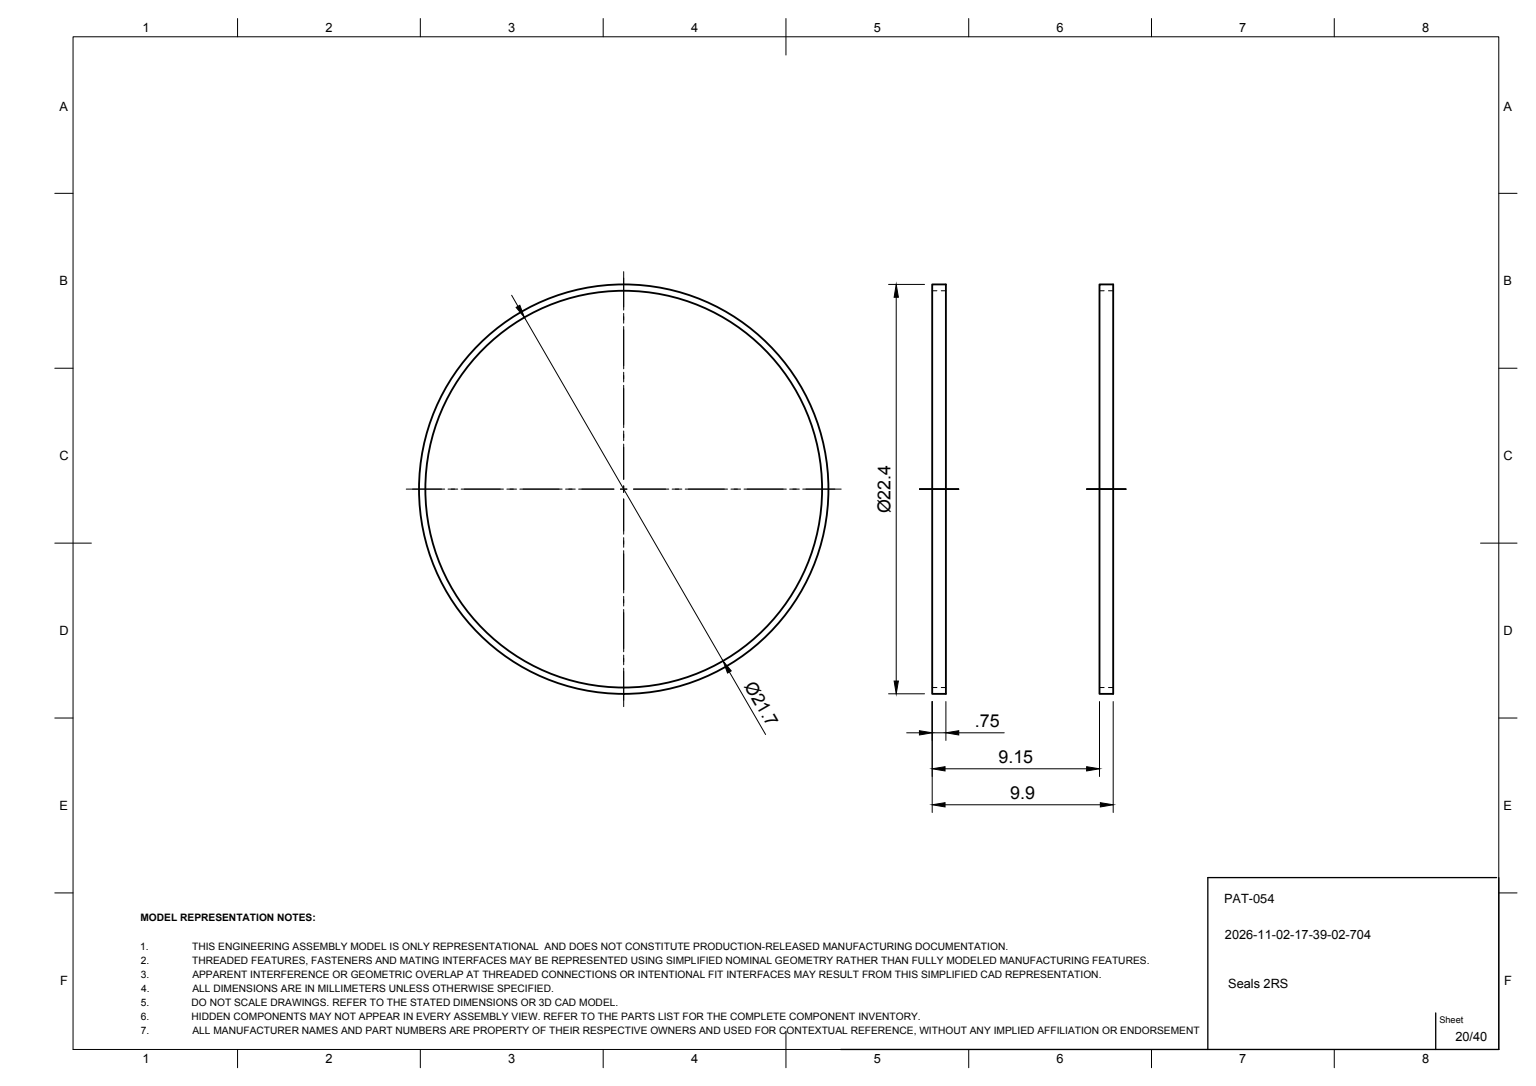
ISO-10303-21;
HEADER;
/* Generated by software containing ST-Developer
 * from STEP Tools, Inc. (www.steptools.com) 
 */

FILE_DESCRIPTION(
/* description */ ('PAT-054'),
/* implementation_level */ '2;1');

FILE_NAME(
/* name */ 'Seals 2RS.step',
/* time_stamp */ '2026-10-29T16:38:13-07:00',
/* author */ (''),
/* organization */ (''),
/* preprocessor_version */ 'ST-DEVELOPER v20.2',
/* originating_system */ 'Autodesk Translation Framework v15.17.0.0',
/* authorisation */ '');

FILE_SCHEMA (('AUTOMOTIVE_DESIGN { 1 0 10303 214 3 1 1 }'));
ENDSEC;

DATA;
#10=MECHANICAL_DESIGN_GEOMETRIC_PRESENTATION_REPRESENTATION('',(#918,#919),#33981);
#824=SHAPE_REPRESENTATION_RELATIONSHIP('SRR','None',#34198,#868);
#868=ADVANCED_BREP_SHAPE_REPRESENTATION('',(#977,#978),#33946);
#918=STYLED_ITEM('',(#34517),#977);
#919=STYLED_ITEM('',(#34517),#978);
#977=MANIFOLD_SOLID_BREP('Body1',#13029);
#978=MANIFOLD_SOLID_BREP('Body2',#13030);
#1133=FACE_BOUND('',#2613,.T.);
#1134=FACE_BOUND('',#2616,.T.);
#1135=FACE_BOUND('',#2619,.T.);
#1136=FACE_BOUND('',#2622,.T.);
#1323=PLANE('',#13978);
#1324=PLANE('',#13983);
#1325=PLANE('',#13986);
#1326=PLANE('',#13991);
#1768=FACE_OUTER_BOUND('',#2612,.T.);
#1769=FACE_OUTER_BOUND('',#2614,.T.);
#1770=FACE_OUTER_BOUND('',#2615,.T.);
#1771=FACE_OUTER_BOUND('',#2617,.T.);
#1772=FACE_OUTER_BOUND('',#2618,.T.);
#1773=FACE_OUTER_BOUND('',#2620,.T.);
#1774=FACE_OUTER_BOUND('',#2621,.T.);
#1775=FACE_OUTER_BOUND('',#2623,.T.);
#2612=EDGE_LOOP('',(#9401));
#2613=EDGE_LOOP('',(#9402));
#2614=EDGE_LOOP('',(#9403,#9404,#9405,#9406));
#2615=EDGE_LOOP('',(#9407));
#2616=EDGE_LOOP('',(#9408));
#2617=EDGE_LOOP('',(#9409,#9410,#9411,#9412));
#2618=EDGE_LOOP('',(#9413));
#2619=EDGE_LOOP('',(#9414));
#2620=EDGE_LOOP('',(#9415,#9416,#9417,#9418));
#2621=EDGE_LOOP('',(#9419));
#2622=EDGE_LOOP('',(#9420));
#2623=EDGE_LOOP('',(#9421,#9422,#9423,#9424));
#3470=LINE('',#19766,#4404);
#3471=LINE('',#19771,#4405);
#3472=LINE('',#19780,#4406);
#3473=LINE('',#19785,#4407);
#4404=VECTOR('',#15971,1.119765);
#4405=VECTOR('',#15978,1.085235);
#4406=VECTOR('',#15989,1.119765);
#4407=VECTOR('',#15996,1.085235);
#5314=CIRCLE('',#13979,1.119765);
#5315=CIRCLE('',#13980,1.085235);
#5316=CIRCLE('',#13982,1.119765);
#5317=CIRCLE('',#13984,1.085235);
#5318=CIRCLE('',#13987,1.119765);
#5319=CIRCLE('',#13988,1.085235);
#5320=CIRCLE('',#13990,1.119765);
#5321=CIRCLE('',#13992,1.085235);
#5882=VERTEX_POINT('',#19759);
#5883=VERTEX_POINT('',#19761);
#5884=VERTEX_POINT('',#19764);
#5885=VERTEX_POINT('',#19768);
#5886=VERTEX_POINT('',#19773);
#5887=VERTEX_POINT('',#19775);
#5888=VERTEX_POINT('',#19778);
#5889=VERTEX_POINT('',#19782);
#7200=EDGE_CURVE('',#5882,#5882,#5314,.T.);
#7201=EDGE_CURVE('',#5883,#5883,#5315,.T.);
#7202=EDGE_CURVE('',#5884,#5884,#5316,.T.);
#7203=EDGE_CURVE('',#5884,#5882,#3470,.T.);
#7204=EDGE_CURVE('',#5885,#5885,#5317,.T.);
#7205=EDGE_CURVE('',#5885,#5883,#3471,.T.);
#7206=EDGE_CURVE('',#5886,#5886,#5318,.T.);
#7207=EDGE_CURVE('',#5887,#5887,#5319,.T.);
#7208=EDGE_CURVE('',#5888,#5888,#5320,.T.);
#7209=EDGE_CURVE('',#5888,#5886,#3472,.T.);
#7210=EDGE_CURVE('',#5889,#5889,#5321,.T.);
#7211=EDGE_CURVE('',#5889,#5887,#3473,.T.);
#9401=ORIENTED_EDGE('',*,*,#7200,.F.);
#9402=ORIENTED_EDGE('',*,*,#7201,.T.);
#9403=ORIENTED_EDGE('',*,*,#7202,.F.);
#9404=ORIENTED_EDGE('',*,*,#7203,.T.);
#9405=ORIENTED_EDGE('',*,*,#7200,.T.);
#9406=ORIENTED_EDGE('',*,*,#7203,.F.);
#9407=ORIENTED_EDGE('',*,*,#7202,.T.);
#9408=ORIENTED_EDGE('',*,*,#7204,.F.);
#9409=ORIENTED_EDGE('',*,*,#7204,.T.);
#9410=ORIENTED_EDGE('',*,*,#7205,.T.);
#9411=ORIENTED_EDGE('',*,*,#7201,.F.);
#9412=ORIENTED_EDGE('',*,*,#7205,.F.);
#9413=ORIENTED_EDGE('',*,*,#7206,.F.);
#9414=ORIENTED_EDGE('',*,*,#7207,.T.);
#9415=ORIENTED_EDGE('',*,*,#7208,.F.);
#9416=ORIENTED_EDGE('',*,*,#7209,.T.);
#9417=ORIENTED_EDGE('',*,*,#7206,.T.);
#9418=ORIENTED_EDGE('',*,*,#7209,.F.);
#9419=ORIENTED_EDGE('',*,*,#7208,.T.);
#9420=ORIENTED_EDGE('',*,*,#7210,.F.);
#9421=ORIENTED_EDGE('',*,*,#7210,.T.);
#9422=ORIENTED_EDGE('',*,*,#7211,.T.);
#9423=ORIENTED_EDGE('',*,*,#7207,.F.);
#9424=ORIENTED_EDGE('',*,*,#7211,.F.);
#12057=CYLINDRICAL_SURFACE('',#13981,1.119765);
#12058=CYLINDRICAL_SURFACE('',#13985,1.085235);
#12059=CYLINDRICAL_SURFACE('',#13989,1.119765);
#12060=CYLINDRICAL_SURFACE('',#13993,1.085235);
#12480=ADVANCED_FACE('',(#1768,#1133),#1323,.T.);
#12481=ADVANCED_FACE('',(#1769),#12057,.T.);
#12482=ADVANCED_FACE('',(#1770,#1134),#1324,.T.);
#12483=ADVANCED_FACE('',(#1771),#12058,.F.);
#12484=ADVANCED_FACE('',(#1772,#1135),#1325,.T.);
#12485=ADVANCED_FACE('',(#1773),#12059,.T.);
#12486=ADVANCED_FACE('',(#1774,#1136),#1326,.T.);
#12487=ADVANCED_FACE('',(#1775),#12060,.F.);
#13029=CLOSED_SHELL('',(#12480,#12481,#12482,#12483));
#13030=CLOSED_SHELL('',(#12484,#12485,#12486,#12487));
#13977=AXIS2_PLACEMENT_3D('',#19757,#15959,#15960);
#13978=AXIS2_PLACEMENT_3D('',#19758,#15961,#15962);
#13979=AXIS2_PLACEMENT_3D('',#19760,#15963,#15964);
#13980=AXIS2_PLACEMENT_3D('',#19762,#15965,#15966);
#13981=AXIS2_PLACEMENT_3D('',#19763,#15967,#15968);
#13982=AXIS2_PLACEMENT_3D('',#19765,#15969,#15970);
#13983=AXIS2_PLACEMENT_3D('',#19767,#15972,#15973);
#13984=AXIS2_PLACEMENT_3D('',#19769,#15974,#15975);
#13985=AXIS2_PLACEMENT_3D('',#19770,#15976,#15977);
#13986=AXIS2_PLACEMENT_3D('',#19772,#15979,#15980);
#13987=AXIS2_PLACEMENT_3D('',#19774,#15981,#15982);
#13988=AXIS2_PLACEMENT_3D('',#19776,#15983,#15984);
#13989=AXIS2_PLACEMENT_3D('',#19777,#15985,#15986);
#13990=AXIS2_PLACEMENT_3D('',#19779,#15987,#15988);
#13991=AXIS2_PLACEMENT_3D('',#19781,#15990,#15991);
#13992=AXIS2_PLACEMENT_3D('',#19783,#15992,#15993);
#13993=AXIS2_PLACEMENT_3D('',#19784,#15994,#15995);
#15959=DIRECTION('axis',(0.,0.,1.));
#15960=DIRECTION('refdir',(1.,0.,0.));
#15961=DIRECTION('center_axis',(0.,1.,0.));
#15962=DIRECTION('ref_axis',(0.,0.,1.));
#15963=DIRECTION('center_axis',(0.,-1.,0.));
#15964=DIRECTION('ref_axis',(1.,0.,0.));
#15965=DIRECTION('center_axis',(0.,-1.,0.));
#15966=DIRECTION('ref_axis',(1.,0.,0.));
#15967=DIRECTION('center_axis',(0.,-1.,0.));
#15968=DIRECTION('ref_axis',(1.,0.,0.));
#15969=DIRECTION('center_axis',(0.,-1.,0.));
#15970=DIRECTION('ref_axis',(1.,0.,0.));
#15971=DIRECTION('',(0.,1.,0.));
#15972=DIRECTION('center_axis',(0.,-1.,0.));
#15973=DIRECTION('ref_axis',(0.,0.,-1.));
#15974=DIRECTION('center_axis',(0.,-1.,0.));
#15975=DIRECTION('ref_axis',(1.,0.,0.));
#15976=DIRECTION('center_axis',(0.,-1.,0.));
#15977=DIRECTION('ref_axis',(1.,0.,0.));
#15978=DIRECTION('',(0.,1.,0.));
#15979=DIRECTION('center_axis',(0.,1.,0.));
#15980=DIRECTION('ref_axis',(0.,0.,1.));
#15981=DIRECTION('center_axis',(0.,-1.,0.));
#15982=DIRECTION('ref_axis',(1.,0.,0.));
#15983=DIRECTION('center_axis',(0.,-1.,0.));
#15984=DIRECTION('ref_axis',(1.,0.,0.));
#15985=DIRECTION('center_axis',(0.,-1.,0.));
#15986=DIRECTION('ref_axis',(1.,0.,0.));
#15987=DIRECTION('center_axis',(0.,-1.,0.));
#15988=DIRECTION('ref_axis',(1.,0.,0.));
#15989=DIRECTION('',(0.,1.,0.));
#15990=DIRECTION('center_axis',(0.,-1.,0.));
#15991=DIRECTION('ref_axis',(0.,0.,-1.));
#15992=DIRECTION('center_axis',(0.,-1.,0.));
#15993=DIRECTION('ref_axis',(1.,0.,0.));
#15994=DIRECTION('center_axis',(0.,-1.,0.));
#15995=DIRECTION('ref_axis',(1.,0.,0.));
#15996=DIRECTION('',(0.,1.,0.));
#19757=CARTESIAN_POINT('',(0.,0.,0.));
#19758=CARTESIAN_POINT('Origin',(1.119765,0.495,0.));
#19759=CARTESIAN_POINT('',(-1.119765,0.495,-1.37131662304724E-16));
#19760=CARTESIAN_POINT('Origin',(0.,0.495,0.));
#19761=CARTESIAN_POINT('',(-1.085235,0.495,-1.32902956907268E-16));
#19762=CARTESIAN_POINT('Origin',(0.,0.495,0.));
#19763=CARTESIAN_POINT('Origin',(0.,0.4575,0.));
#19764=CARTESIAN_POINT('',(-1.119765,0.42,-1.37131662304724E-16));
#19765=CARTESIAN_POINT('Origin',(0.,0.42,0.));
#19766=CARTESIAN_POINT('',(-1.119765,0.4575,-1.37131662304724E-16));
#19767=CARTESIAN_POINT('Origin',(1.085235,0.42,0.));
#19768=CARTESIAN_POINT('',(-1.085235,0.42,-1.32902956907268E-16));
#19769=CARTESIAN_POINT('Origin',(0.,0.42,0.));
#19770=CARTESIAN_POINT('Origin',(0.,0.4575,0.));
#19771=CARTESIAN_POINT('',(-1.085235,0.4575,-1.32902956907268E-16));
#19772=CARTESIAN_POINT('Origin',(1.119765,-0.42,0.));
#19773=CARTESIAN_POINT('',(-1.119765,-0.42,-1.37131662304724E-16));
#19774=CARTESIAN_POINT('Origin',(0.,-0.42,0.));
#19775=CARTESIAN_POINT('',(-1.085235,-0.42,-1.32902956907268E-16));
#19776=CARTESIAN_POINT('Origin',(0.,-0.42,0.));
#19777=CARTESIAN_POINT('Origin',(0.,-0.4575,0.));
#19778=CARTESIAN_POINT('',(-1.119765,-0.495,-1.37131662304724E-16));
#19779=CARTESIAN_POINT('Origin',(0.,-0.495,0.));
#19780=CARTESIAN_POINT('',(-1.119765,-0.4575,-1.37131662304724E-16));
#19781=CARTESIAN_POINT('Origin',(1.085235,-0.495,0.));
#19782=CARTESIAN_POINT('',(-1.085235,-0.495,-1.32902956907268E-16));
#19783=CARTESIAN_POINT('Origin',(0.,-0.495,0.));
#19784=CARTESIAN_POINT('Origin',(0.,-0.4575,0.));
#19785=CARTESIAN_POINT('',(-1.085235,-0.4575,-1.32902956907268E-16));
#33894=UNCERTAINTY_MEASURE_WITH_UNIT(LENGTH_MEASURE(0.001),#33982,
'DISTANCE_ACCURACY_VALUE',
'Maximum model space distance between geometric entities at asserted c
onnectivities');
#33929=UNCERTAINTY_MEASURE_WITH_UNIT(LENGTH_MEASURE(0.001),#33982,
'DISTANCE_ACCURACY_VALUE',
'Maximum model space distance between geometric entities at asserted c
onnectivities');
#33946=(
GEOMETRIC_REPRESENTATION_CONTEXT(3)
GLOBAL_UNCERTAINTY_ASSIGNED_CONTEXT((#33894))
GLOBAL_UNIT_ASSIGNED_CONTEXT((#33982,#33984,#33985))
REPRESENTATION_CONTEXT('','3D')
);
#33981=(
GEOMETRIC_REPRESENTATION_CONTEXT(3)
GLOBAL_UNCERTAINTY_ASSIGNED_CONTEXT((#33929))
GLOBAL_UNIT_ASSIGNED_CONTEXT((#33982,#33984,#33985))
REPRESENTATION_CONTEXT('','3D')
);
#33982=(
LENGTH_UNIT()
NAMED_UNIT(*)
SI_UNIT(.CENTI.,.METRE.)
);
#33984=(
NAMED_UNIT(*)
PLANE_ANGLE_UNIT()
SI_UNIT($,.RADIAN.)
);
#33985=(
NAMED_UNIT(*)
SI_UNIT($,.STERADIAN.)
SOLID_ANGLE_UNIT()
);
#34002=SHAPE_DEFINITION_REPRESENTATION(#34053,#34198);
#34053=PRODUCT_DEFINITION_SHAPE('',$,#34250);
#34198=SHAPE_REPRESENTATION('',(#13977),#33946);
#34233=PRODUCT_DEFINITION_CONTEXT('part definition',#34388,'design');
#34250=PRODUCT_DEFINITION('Seals 2RS','Seals 2RS',#34301,#34233);
#34301=PRODUCT_DEFINITION_FORMATION('',$,#34406);
#34388=APPLICATION_CONTEXT(
'Core Data for Automotive Mechanical Design Process');
#34389=PRODUCT_CONTEXT('part definition',#34388,'mechanical');
#34406=PRODUCT('Seals 2RS','Seals 2RS','Seals 2RS',(#34389));
#34511=COLOUR_RGB('Grey',0.48,0.52,0.57);
#34512=FILL_AREA_STYLE_COLOUR('',#34511);
#34513=FILL_AREA_STYLE('',(#34512));
#34514=SURFACE_STYLE_FILL_AREA(#34513);
#34515=SURFACE_SIDE_STYLE('',(#34514));
#34516=SURFACE_STYLE_USAGE(.BOTH.,#34515);
#34517=PRESENTATION_STYLE_ASSIGNMENT((#34516));
ENDSEC;
END-ISO-10303-21;
